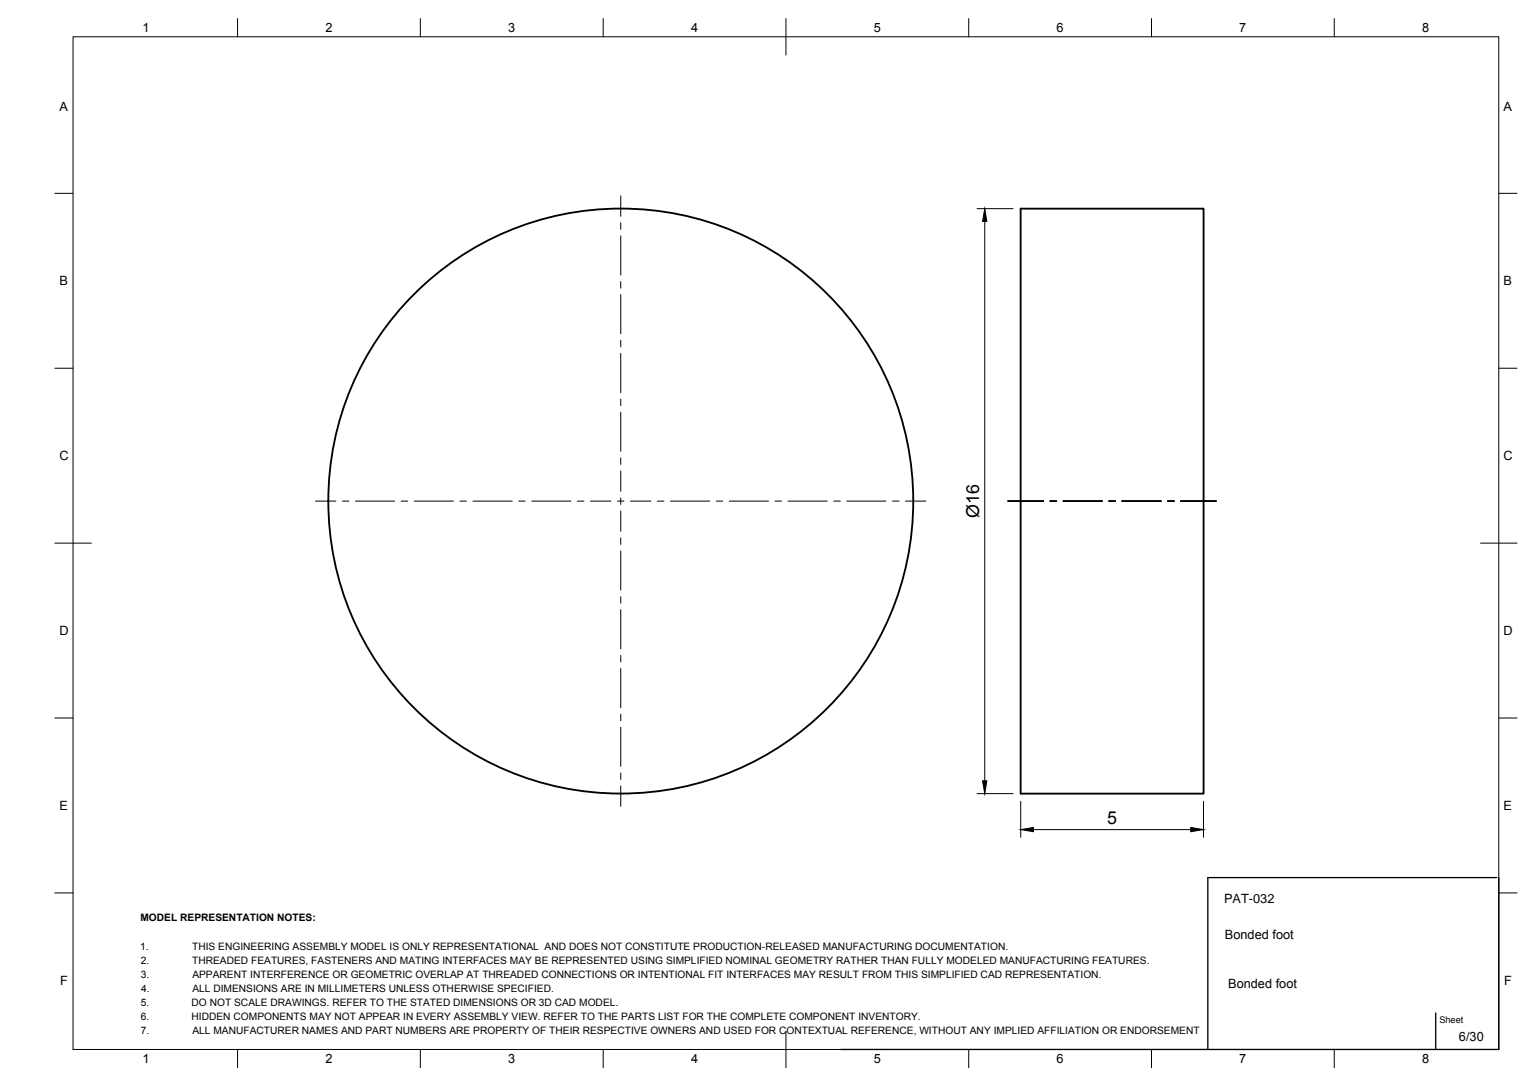
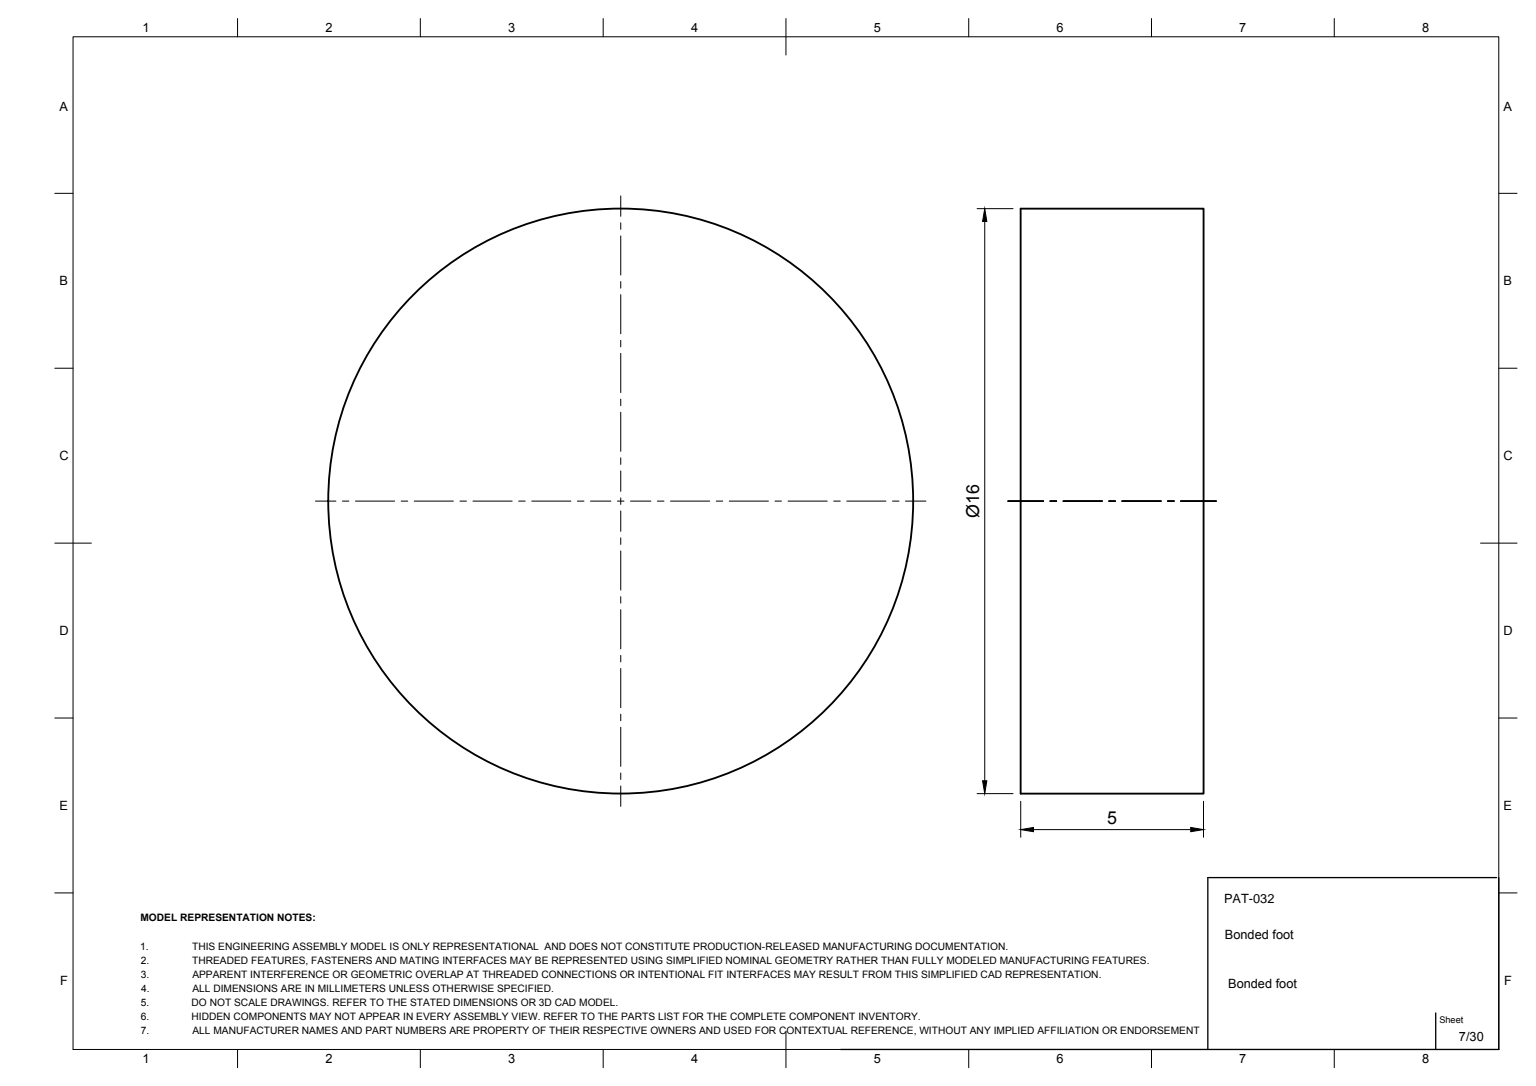
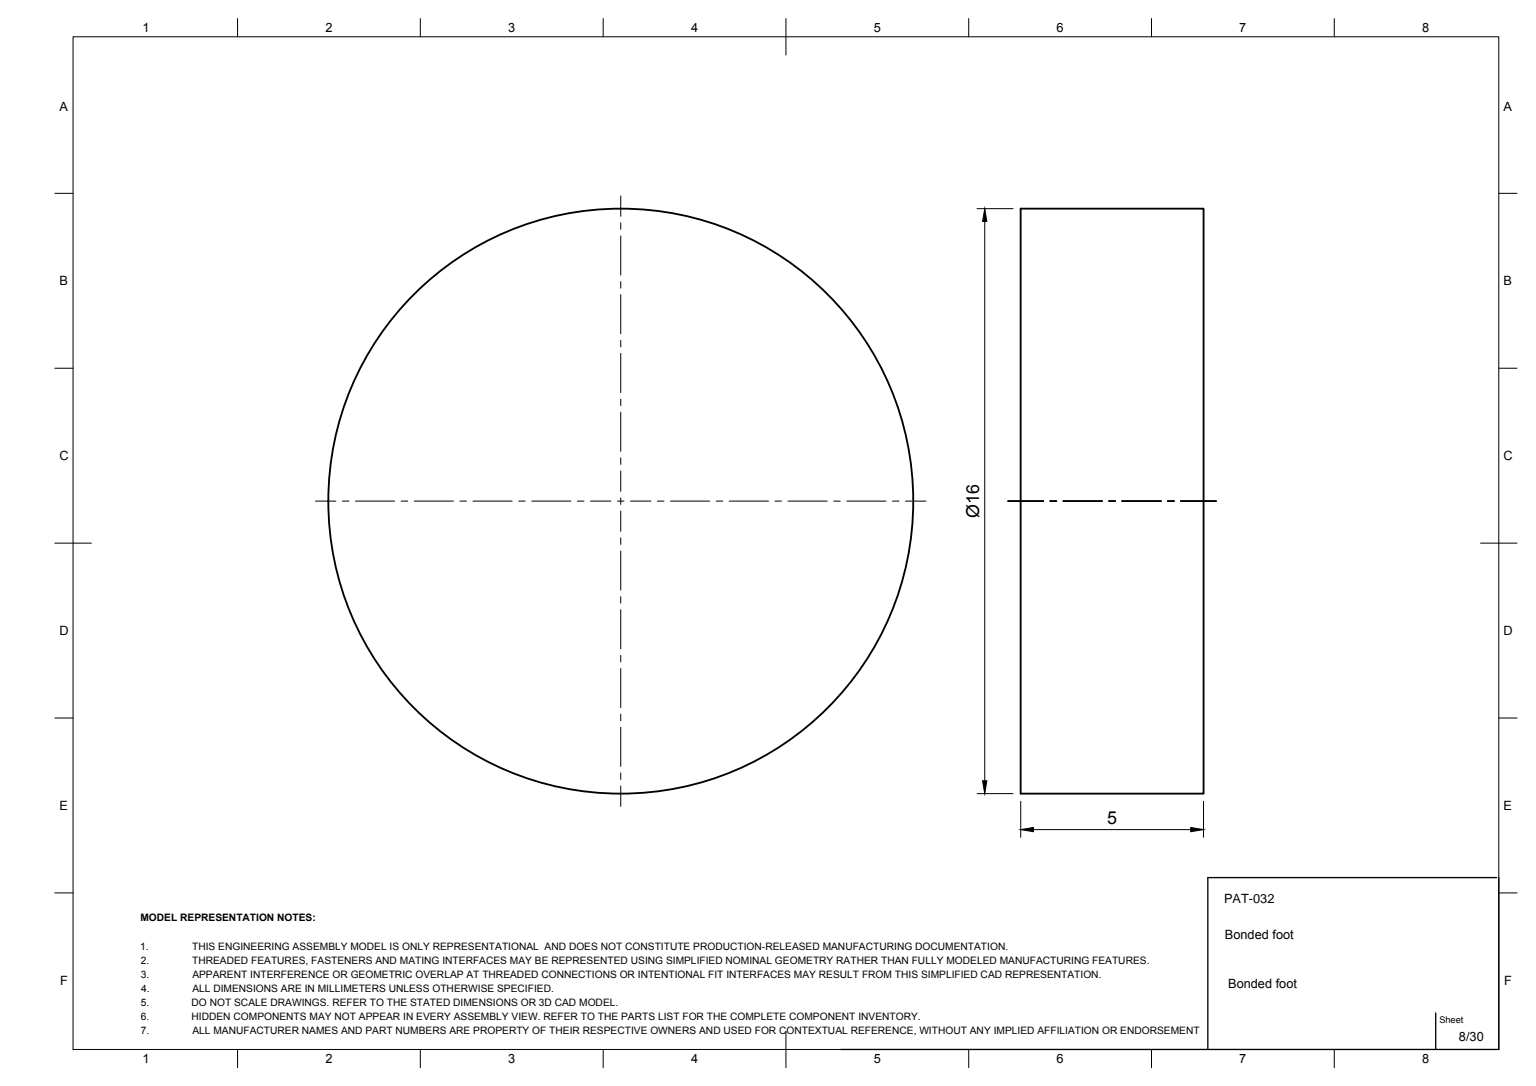
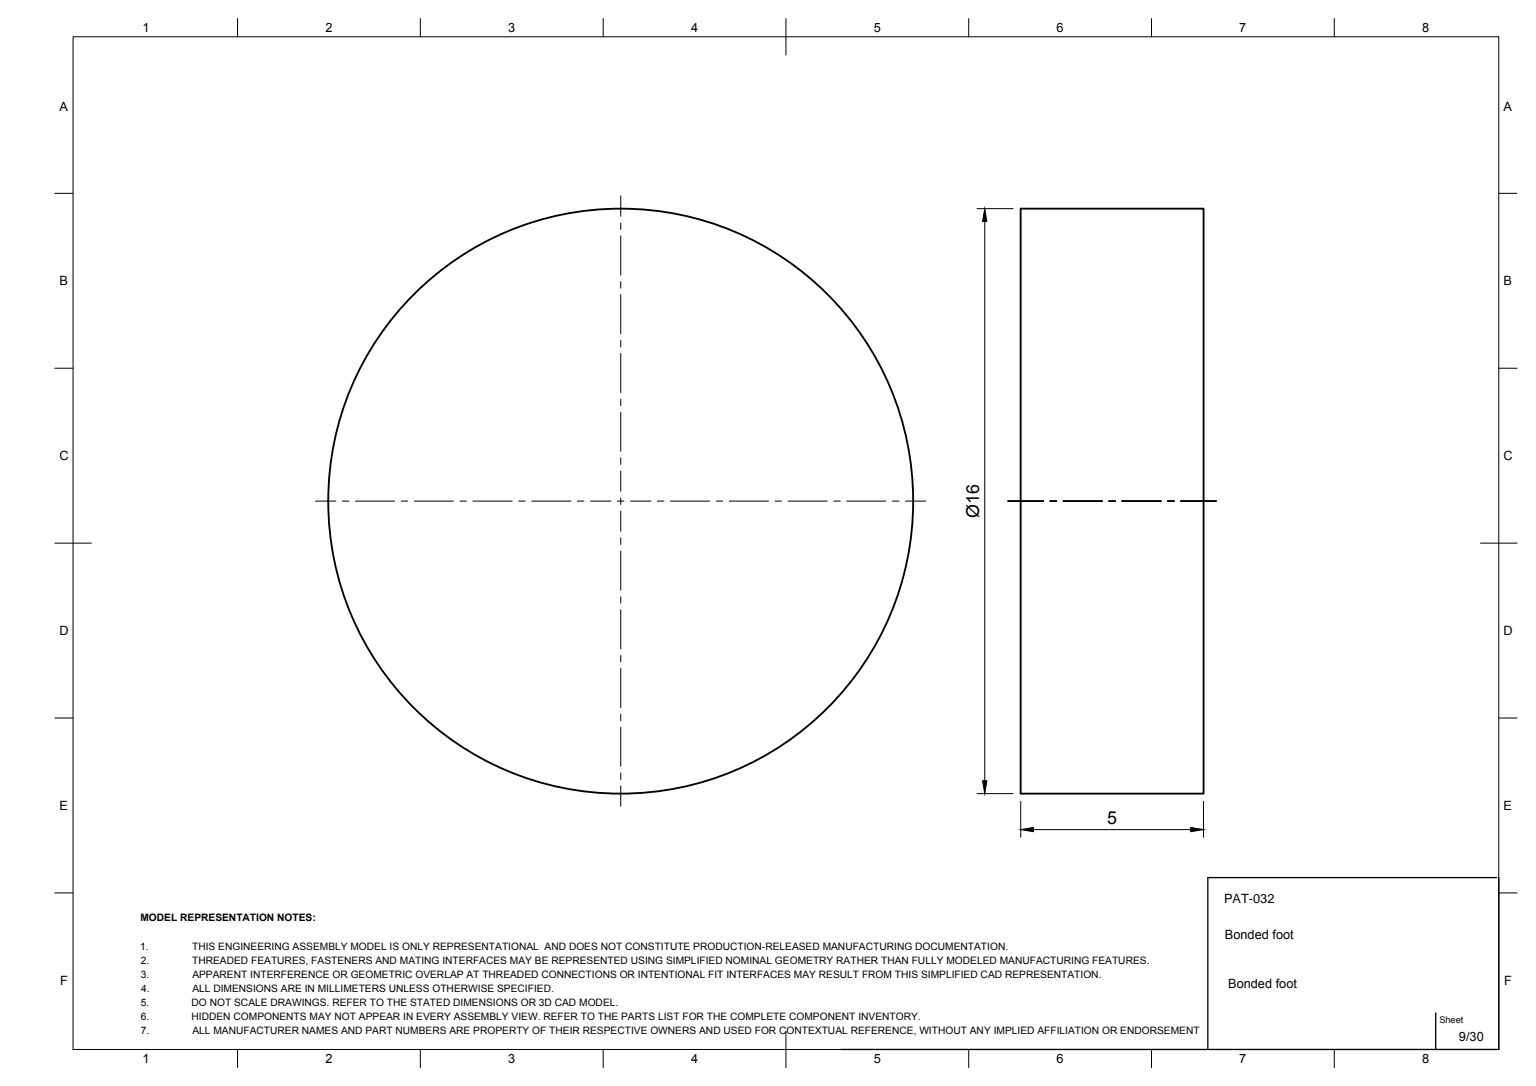
ISO-10303-21;
HEADER;
/* Generated by software containing ST-Developer
 * from STEP Tools, Inc. (www.steptools.com) 
 */

FILE_DESCRIPTION(
/* description */ ('Drill jig with bushing plate'),
/* implementation_level */ '2;1');

FILE_NAME(
/* name */ 'Bonded foot.step',
/* time_stamp */ '2026-10-27T10:51:08-07:00',
/* author */ (''),
/* organization */ (''),
/* preprocessor_version */ 'ST-DEVELOPER v20.2',
/* originating_system */ 'Autodesk Translation Framework v15.17.0.0',
/* authorisation */ '');

FILE_SCHEMA (('AUTOMOTIVE_DESIGN { 1 0 10303 214 3 1 1 }'));
ENDSEC;

DATA;
#10=MECHANICAL_DESIGN_GEOMETRIC_PRESENTATION_REPRESENTATION('',(#224),#6638);
#176=SHAPE_REPRESENTATION_RELATIONSHIP('SRR','None',#6740,#200);
#200=ADVANCED_BREP_SHAPE_REPRESENTATION('',(#248),#6613);
#224=STYLED_ITEM('',(#6957),#248);
#248=MANIFOLD_SOLID_BREP('Body1',#3591);
#376=PLANE('',#3936);
#377=PLANE('',#3937);
#521=FACE_OUTER_BOUND('',#763,.T.);
#522=FACE_OUTER_BOUND('',#764,.T.);
#523=FACE_OUTER_BOUND('',#765,.T.);
#763=EDGE_LOOP('',(#2545,#2546,#2547,#2548));
#764=EDGE_LOOP('',(#2549));
#765=EDGE_LOOP('',(#2550));
#1056=LINE('',#5604,#1317);
#1317=VECTOR('',#4463,0.800000000000001);
#1580=CIRCLE('',#3934,0.800000000000001);
#1581=CIRCLE('',#3935,0.800000000000001);
#1756=VERTEX_POINT('',#5601);
#1757=VERTEX_POINT('',#5603);
#2060=EDGE_CURVE('',#1756,#1756,#1580,.T.);
#2061=EDGE_CURVE('',#1756,#1757,#1056,.T.);
#2062=EDGE_CURVE('',#1757,#1757,#1581,.T.);
#2545=ORIENTED_EDGE('',*,*,#2060,.F.);
#2546=ORIENTED_EDGE('',*,*,#2061,.T.);
#2547=ORIENTED_EDGE('',*,*,#2062,.T.);
#2548=ORIENTED_EDGE('',*,*,#2061,.F.);
#2549=ORIENTED_EDGE('',*,*,#2060,.T.);
#2550=ORIENTED_EDGE('',*,*,#2062,.F.);
#3313=CYLINDRICAL_SURFACE('',#3933,0.800000000000001);
#3396=ADVANCED_FACE('',(#521),#3313,.T.);
#3397=ADVANCED_FACE('',(#522),#376,.T.);
#3398=ADVANCED_FACE('',(#523),#377,.F.);
#3591=CLOSED_SHELL('',(#3396,#3397,#3398));
#3932=AXIS2_PLACEMENT_3D('',#5599,#4457,#4458);
#3933=AXIS2_PLACEMENT_3D('',#5600,#4459,#4460);
#3934=AXIS2_PLACEMENT_3D('',#5602,#4461,#4462);
#3935=AXIS2_PLACEMENT_3D('',#5605,#4464,#4465);
#3936=AXIS2_PLACEMENT_3D('',#5606,#4466,#4467);
#3937=AXIS2_PLACEMENT_3D('',#5607,#4468,#4469);
#4457=DIRECTION('axis',(0.,0.,1.));
#4458=DIRECTION('refdir',(1.,0.,0.));
#4459=DIRECTION('center_axis',(0.,0.,1.));
#4460=DIRECTION('ref_axis',(1.,0.,0.));
#4461=DIRECTION('center_axis',(0.,0.,1.));
#4462=DIRECTION('ref_axis',(1.,0.,0.));
#4463=DIRECTION('',(0.,0.,-1.));
#4464=DIRECTION('center_axis',(0.,0.,1.));
#4465=DIRECTION('ref_axis',(1.,0.,0.));
#4466=DIRECTION('center_axis',(0.,0.,1.));
#4467=DIRECTION('ref_axis',(1.,0.,0.));
#4468=DIRECTION('center_axis',(0.,0.,1.));
#4469=DIRECTION('ref_axis',(1.,0.,0.));
#5599=CARTESIAN_POINT('',(0.,0.,0.));
#5600=CARTESIAN_POINT('Origin',(-9.,-7.,-0.5));
#5601=CARTESIAN_POINT('',(-9.8,-7.,0.));
#5602=CARTESIAN_POINT('Origin',(-9.,-7.,0.));
#5603=CARTESIAN_POINT('',(-9.8,-7.,-0.5));
#5604=CARTESIAN_POINT('',(-9.8,-7.,-0.5));
#5605=CARTESIAN_POINT('Origin',(-9.,-7.,-0.5));
#5606=CARTESIAN_POINT('Origin',(-9.,-7.,0.));
#5607=CARTESIAN_POINT('Origin',(-9.,-7.,-0.5));
#6584=UNCERTAINTY_MEASURE_WITH_UNIT(LENGTH_MEASURE(0.001),#6639,
'DISTANCE_ACCURACY_VALUE',
'Maximum model space distance between geometric entities at asserted c
onnectivities');
#6609=UNCERTAINTY_MEASURE_WITH_UNIT(LENGTH_MEASURE(0.001),#6639,
'DISTANCE_ACCURACY_VALUE',
'Maximum model space distance between geometric entities at asserted c
onnectivities');
#6613=(
GEOMETRIC_REPRESENTATION_CONTEXT(3)
GLOBAL_UNCERTAINTY_ASSIGNED_CONTEXT((#6584))
GLOBAL_UNIT_ASSIGNED_CONTEXT((#6639,#6641,#6642))
REPRESENTATION_CONTEXT('','3D')
);
#6638=(
GEOMETRIC_REPRESENTATION_CONTEXT(3)
GLOBAL_UNCERTAINTY_ASSIGNED_CONTEXT((#6609))
GLOBAL_UNIT_ASSIGNED_CONTEXT((#6639,#6641,#6642))
REPRESENTATION_CONTEXT('','3D')
);
#6639=(
LENGTH_UNIT()
NAMED_UNIT(*)
SI_UNIT(.CENTI.,.METRE.)
);
#6641=(
NAMED_UNIT(*)
PLANE_ANGLE_UNIT()
SI_UNIT($,.RADIAN.)
);
#6642=(
NAMED_UNIT(*)
SI_UNIT($,.STERADIAN.)
SOLID_ANGLE_UNIT()
);
#6646=SHAPE_DEFINITION_REPRESENTATION(#6674,#6740);
#6674=PRODUCT_DEFINITION_SHAPE('',$,#6769);
#6740=SHAPE_REPRESENTATION('',(#3932),#6613);
#6765=PRODUCT_DEFINITION_CONTEXT('part definition',#6851,'design');
#6769=PRODUCT_DEFINITION('Bonded foot','Bonded foot',#6797,#6765);
#6797=PRODUCT_DEFINITION_FORMATION('',$,#6856);
#6851=APPLICATION_CONTEXT(
'Core Data for Automotive Mechanical Design Process');
#6852=PRODUCT_CONTEXT('part definition',#6851,'mechanical');
#6856=PRODUCT('Bonded foot','Bonded foot','Bonded foot',(#6852));
#6951=COLOUR_RGB('Off White',0.89,0.88,0.83);
#6952=FILL_AREA_STYLE_COLOUR('',#6951);
#6953=FILL_AREA_STYLE('',(#6952));
#6954=SURFACE_STYLE_FILL_AREA(#6953);
#6955=SURFACE_SIDE_STYLE('',(#6954));
#6956=SURFACE_STYLE_USAGE(.BOTH.,#6955);
#6957=PRESENTATION_STYLE_ASSIGNMENT((#6956));
ENDSEC;
END-ISO-10303-21;
